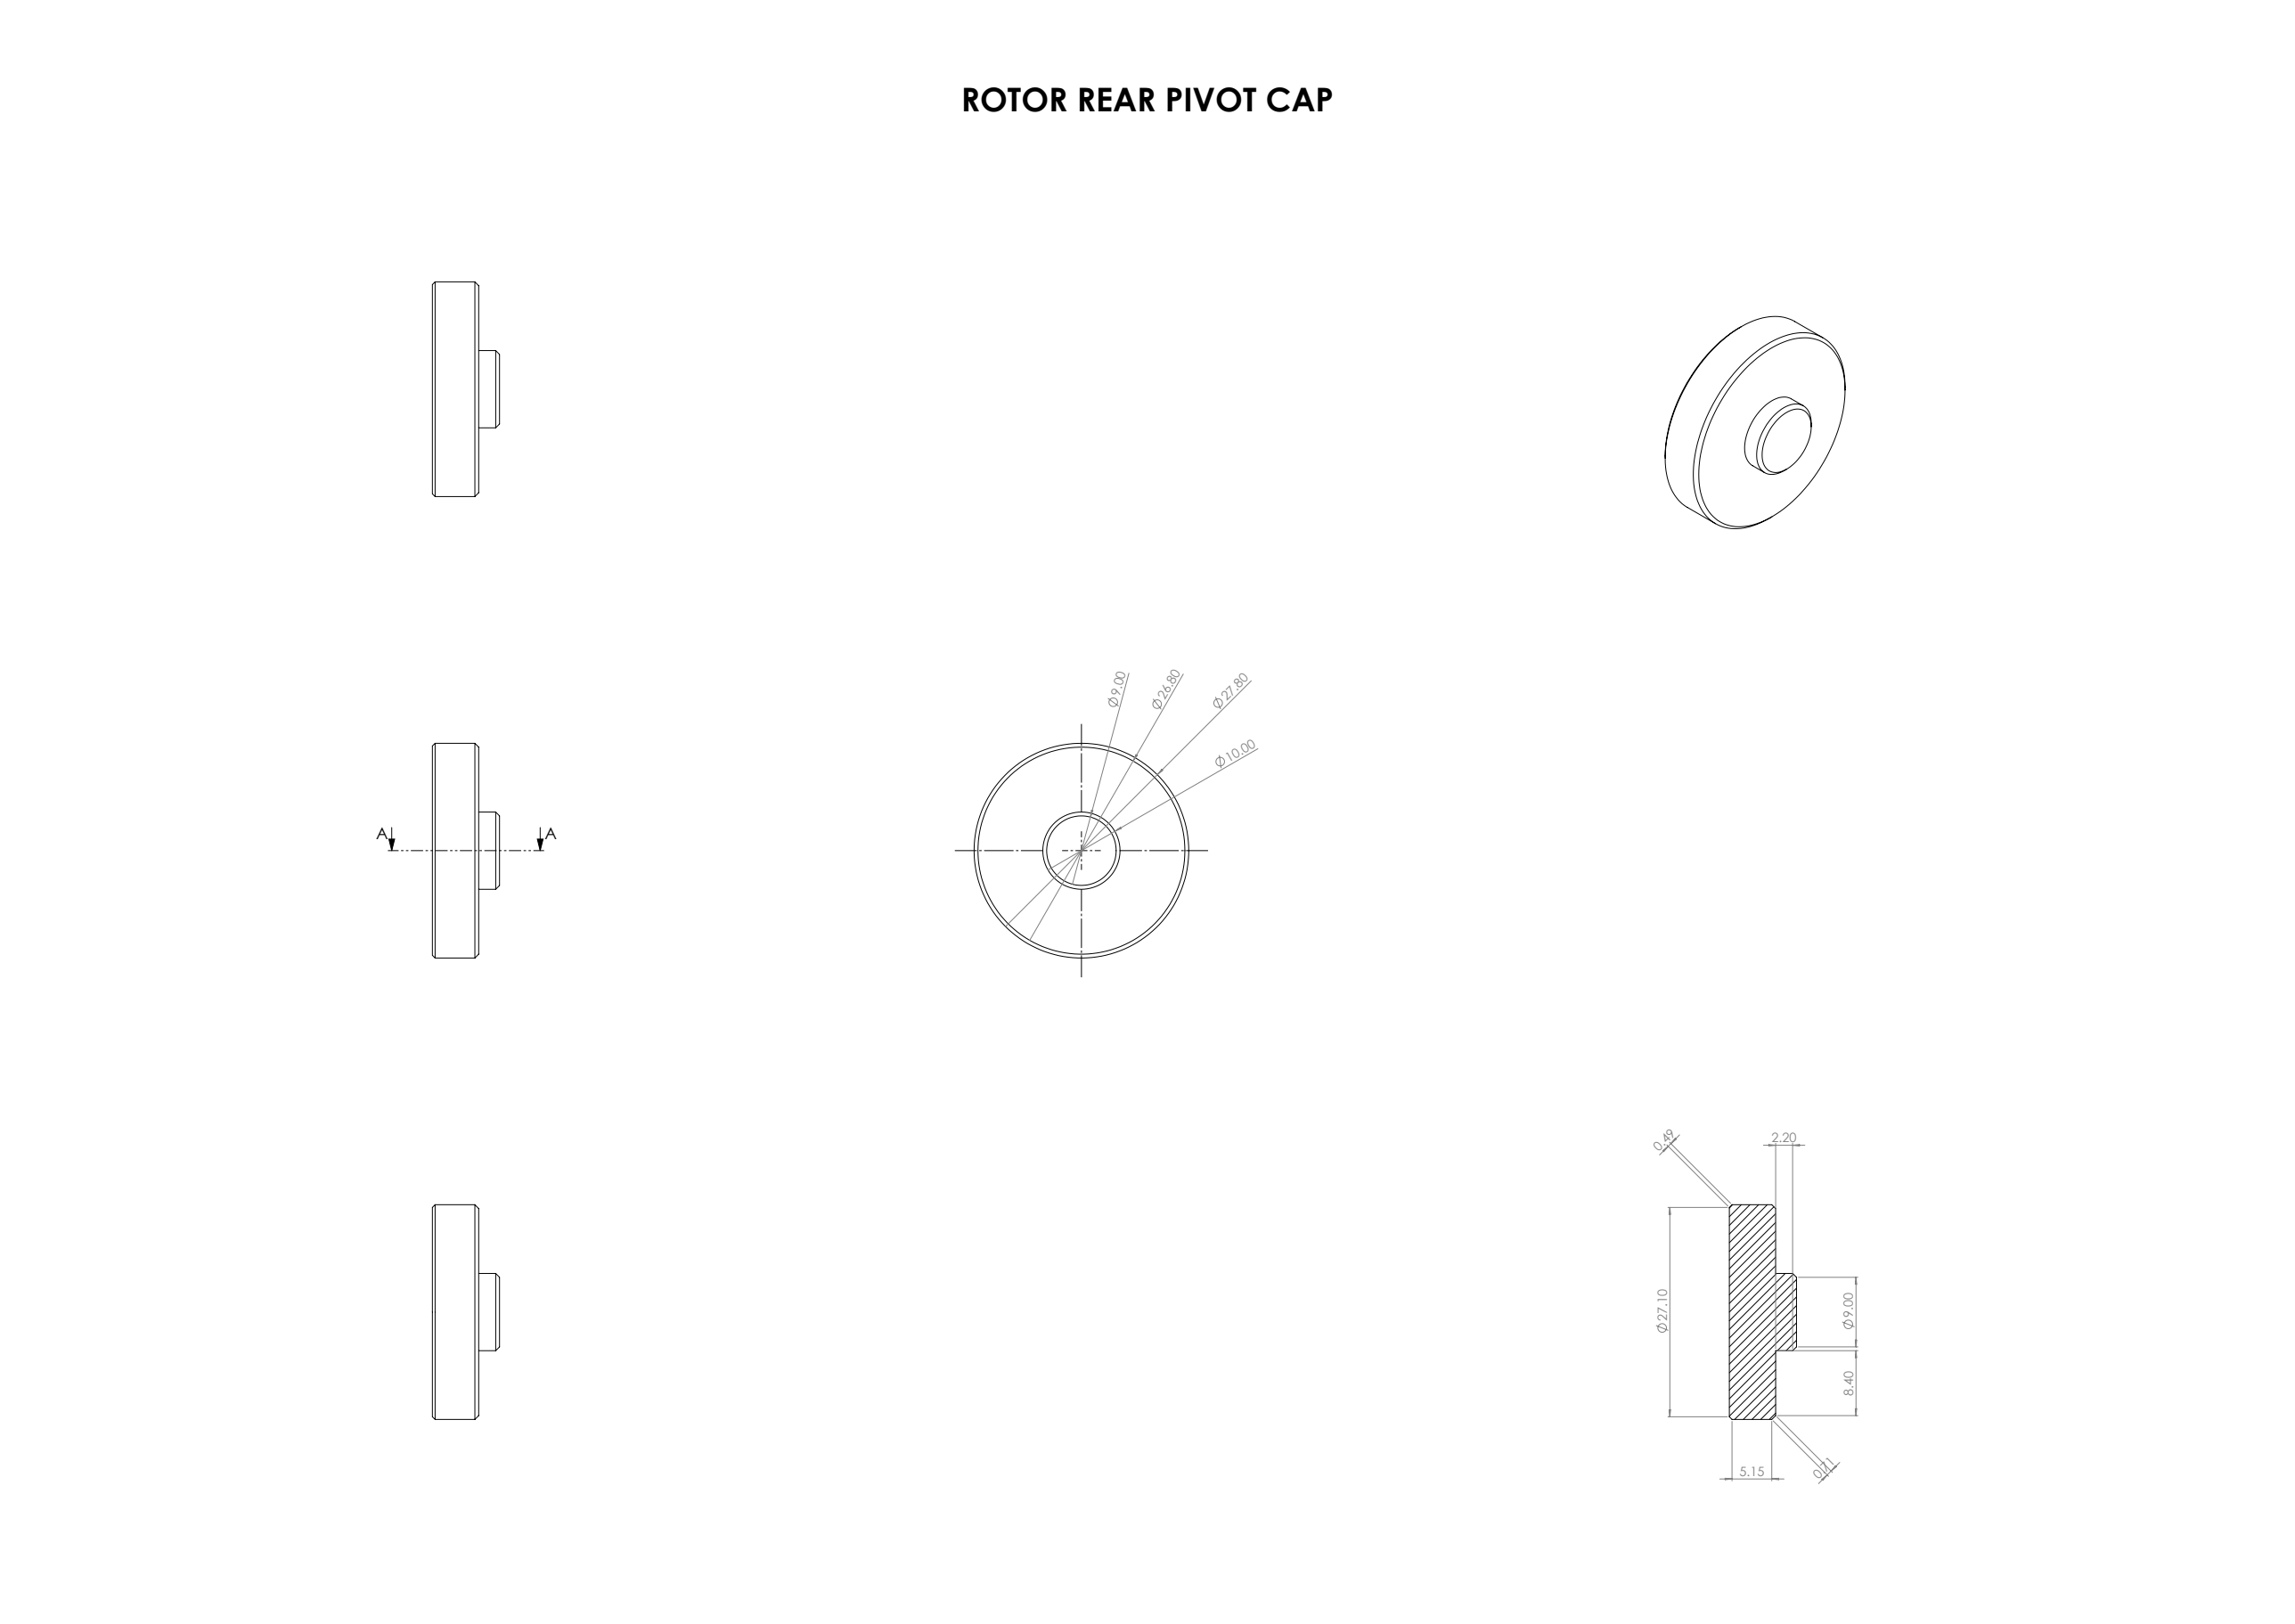
ISO-10303-21;
HEADER;
/* Generated by software containing ST-Developer
 * from STEP Tools, Inc. (www.steptools.com) 
 */

FILE_DESCRIPTION(
/* description */ (''),
/* implementation_level */ '2;1');

FILE_NAME(
/* name */ '05_Rotor_Rear_Pivot_Cap.step',
/* time_stamp */ '2026-10-21T01:59:45-07:00',
/* author */ (''),
/* organization */ (''),
/* preprocessor_version */ 'ST-DEVELOPER v20.2',
/* originating_system */ 'Autodesk Translation Framework v15.15.0.0',
/* authorisation */ '');

FILE_SCHEMA (('AUTOMOTIVE_DESIGN { 1 0 10303 214 3 1 1 }'));
ENDSEC;

DATA;
#10=MECHANICAL_DESIGN_GEOMETRIC_PRESENTATION_REPRESENTATION('',(#475),#18281);
#417=CONICAL_SURFACE('',#9697,13.725,0.785398163397447);
#418=CONICAL_SURFACE('',#9704,13.65,0.78539816339745);
#419=CONICAL_SURFACE('',#9710,4.75,0.785398163397449);
#444=SHAPE_REPRESENTATION_RELATIONSHIP('SRR','None',#18346,#457);
#457=ADVANCED_BREP_SHAPE_REPRESENTATION('',(#488),#18275);
#475=STYLED_ITEM('',(#18488),#488);
#488=MANIFOLD_SOLID_BREP('Body1',#9092);
#528=CYLINDRICAL_SURFACE('',#9702,13.9);
#529=CYLINDRICAL_SURFACE('',#9708,5.);
#619=FACE_BOUND('',#1765,.T.);
#747=CIRCLE('',#9698,13.9);
#748=CIRCLE('',#9699,13.9);
#749=CIRCLE('',#9700,13.55);
#750=CIRCLE('',#9703,13.9);
#751=CIRCLE('',#9705,13.4);
#752=CIRCLE('',#9707,5.);
#753=CIRCLE('',#9709,5.);
#754=CIRCLE('',#9711,4.5);
#1198=FACE_OUTER_BOUND('',#1760,.T.);
#1199=FACE_OUTER_BOUND('',#1761,.T.);
#1200=FACE_OUTER_BOUND('',#1762,.T.);
#1201=FACE_OUTER_BOUND('',#1763,.T.);
#1202=FACE_OUTER_BOUND('',#1764,.T.);
#1203=FACE_OUTER_BOUND('',#1766,.T.);
#1204=FACE_OUTER_BOUND('',#1767,.T.);
#1205=FACE_OUTER_BOUND('',#1768,.T.);
#1760=EDGE_LOOP('',(#7414,#7415,#7416,#7417,#7418));
#1761=EDGE_LOOP('',(#7419));
#1762=EDGE_LOOP('',(#7420,#7421,#7422,#7423,#7424));
#1763=EDGE_LOOP('',(#7425,#7426,#7427,#7428));
#1764=EDGE_LOOP('',(#7429));
#1765=EDGE_LOOP('',(#7430));
#1766=EDGE_LOOP('',(#7431,#7432,#7433,#7434));
#1767=EDGE_LOOP('',(#7435,#7436,#7437,#7438));
#1768=EDGE_LOOP('',(#7439));
#2562=LINE('',#14511,#3407);
#2563=LINE('',#14517,#3408);
#2564=LINE('',#14521,#3409);
#2565=LINE('',#14528,#3410);
#2566=LINE('',#14532,#3411);
#3407=VECTOR('',#11512,13.725);
#3408=VECTOR('',#11521,13.9);
#3409=VECTOR('',#11526,13.65);
#3410=VECTOR('',#11535,5.);
#3411=VECTOR('',#11540,4.75);
#4153=VERTEX_POINT('',#14506);
#4154=VERTEX_POINT('',#14507);
#4155=VERTEX_POINT('',#14510);
#4156=VERTEX_POINT('',#14515);
#4157=VERTEX_POINT('',#14519);
#4158=VERTEX_POINT('',#14523);
#4159=VERTEX_POINT('',#14526);
#4160=VERTEX_POINT('',#14530);
#5279=EDGE_CURVE('',#4153,#4154,#747,.T.);
#5280=EDGE_CURVE('',#4154,#4153,#748,.T.);
#5281=EDGE_CURVE('',#4153,#4155,#2562,.T.);
#5282=EDGE_CURVE('',#4155,#4155,#749,.T.);
#5283=EDGE_CURVE('',#4156,#4156,#750,.T.);
#5284=EDGE_CURVE('',#4156,#4154,#2563,.T.);
#5285=EDGE_CURVE('',#4157,#4157,#751,.T.);
#5286=EDGE_CURVE('',#4157,#4156,#2564,.T.);
#5287=EDGE_CURVE('',#4158,#4158,#752,.T.);
#5288=EDGE_CURVE('',#4159,#4159,#753,.T.);
#5289=EDGE_CURVE('',#4159,#4158,#2565,.T.);
#5290=EDGE_CURVE('',#4160,#4160,#754,.T.);
#5291=EDGE_CURVE('',#4160,#4159,#2566,.T.);
#7414=ORIENTED_EDGE('',*,*,#5279,.T.);
#7415=ORIENTED_EDGE('',*,*,#5280,.T.);
#7416=ORIENTED_EDGE('',*,*,#5281,.T.);
#7417=ORIENTED_EDGE('',*,*,#5282,.T.);
#7418=ORIENTED_EDGE('',*,*,#5281,.F.);
#7419=ORIENTED_EDGE('',*,*,#5282,.F.);
#7420=ORIENTED_EDGE('',*,*,#5283,.F.);
#7421=ORIENTED_EDGE('',*,*,#5284,.T.);
#7422=ORIENTED_EDGE('',*,*,#5279,.F.);
#7423=ORIENTED_EDGE('',*,*,#5280,.F.);
#7424=ORIENTED_EDGE('',*,*,#5284,.F.);
#7425=ORIENTED_EDGE('',*,*,#5285,.F.);
#7426=ORIENTED_EDGE('',*,*,#5286,.T.);
#7427=ORIENTED_EDGE('',*,*,#5283,.T.);
#7428=ORIENTED_EDGE('',*,*,#5286,.F.);
#7429=ORIENTED_EDGE('',*,*,#5285,.T.);
#7430=ORIENTED_EDGE('',*,*,#5287,.F.);
#7431=ORIENTED_EDGE('',*,*,#5288,.F.);
#7432=ORIENTED_EDGE('',*,*,#5289,.T.);
#7433=ORIENTED_EDGE('',*,*,#5287,.T.);
#7434=ORIENTED_EDGE('',*,*,#5289,.F.);
#7435=ORIENTED_EDGE('',*,*,#5290,.F.);
#7436=ORIENTED_EDGE('',*,*,#5291,.T.);
#7437=ORIENTED_EDGE('',*,*,#5288,.T.);
#7438=ORIENTED_EDGE('',*,*,#5291,.F.);
#7439=ORIENTED_EDGE('',*,*,#5290,.T.);
#8473=PLANE('',#9701);
#8474=PLANE('',#9706);
#8475=PLANE('',#9712);
#8919=ADVANCED_FACE('',(#1198),#417,.T.);
#8920=ADVANCED_FACE('',(#1199),#8473,.T.);
#8921=ADVANCED_FACE('',(#1200),#528,.T.);
#8922=ADVANCED_FACE('',(#1201),#418,.T.);
#8923=ADVANCED_FACE('',(#1202,#619),#8474,.T.);
#8924=ADVANCED_FACE('',(#1203),#529,.T.);
#8925=ADVANCED_FACE('',(#1204),#419,.T.);
#8926=ADVANCED_FACE('',(#1205),#8475,.T.);
#9092=CLOSED_SHELL('',(#8919,#8920,#8921,#8922,#8923,#8924,#8925,#8926));
#9696=AXIS2_PLACEMENT_3D('',#14504,#11504,#11505);
#9697=AXIS2_PLACEMENT_3D('',#14505,#11506,#11507);
#9698=AXIS2_PLACEMENT_3D('',#14508,#11508,#11509);
#9699=AXIS2_PLACEMENT_3D('',#14509,#11510,#11511);
#9700=AXIS2_PLACEMENT_3D('',#14512,#11513,#11514);
#9701=AXIS2_PLACEMENT_3D('',#14513,#11515,#11516);
#9702=AXIS2_PLACEMENT_3D('',#14514,#11517,#11518);
#9703=AXIS2_PLACEMENT_3D('',#14516,#11519,#11520);
#9704=AXIS2_PLACEMENT_3D('',#14518,#11522,#11523);
#9705=AXIS2_PLACEMENT_3D('',#14520,#11524,#11525);
#9706=AXIS2_PLACEMENT_3D('',#14522,#11527,#11528);
#9707=AXIS2_PLACEMENT_3D('',#14524,#11529,#11530);
#9708=AXIS2_PLACEMENT_3D('',#14525,#11531,#11532);
#9709=AXIS2_PLACEMENT_3D('',#14527,#11533,#11534);
#9710=AXIS2_PLACEMENT_3D('',#14529,#11536,#11537);
#9711=AXIS2_PLACEMENT_3D('',#14531,#11538,#11539);
#9712=AXIS2_PLACEMENT_3D('',#14533,#11541,#11542);
#11504=DIRECTION('axis',(0.,0.,1.));
#11505=DIRECTION('refdir',(1.,0.,0.));
#11506=DIRECTION('center_axis',(1.,0.,0.));
#11507=DIRECTION('ref_axis',(0.,-1.,0.));
#11508=DIRECTION('center_axis',(-1.,0.,0.));
#11509=DIRECTION('ref_axis',(0.,-1.,0.));
#11510=DIRECTION('center_axis',(-1.,0.,0.));
#11511=DIRECTION('ref_axis',(0.,-1.,0.));
#11512=DIRECTION('',(-0.707106781186548,-0.707106781186547,-8.65956056235492E-17));
#11513=DIRECTION('center_axis',(1.,0.,0.));
#11514=DIRECTION('ref_axis',(0.,-1.,0.));
#11515=DIRECTION('center_axis',(-1.,0.,0.));
#11516=DIRECTION('ref_axis',(0.,0.,1.));
#11517=DIRECTION('center_axis',(1.,0.,0.));
#11518=DIRECTION('ref_axis',(0.,1.,0.));
#11519=DIRECTION('center_axis',(1.,0.,0.));
#11520=DIRECTION('ref_axis',(0.,0.,-1.));
#11521=DIRECTION('',(-1.,0.,0.));
#11522=DIRECTION('center_axis',(-1.,0.,0.));
#11523=DIRECTION('ref_axis',(0.,1.,0.));
#11524=DIRECTION('center_axis',(1.,0.,0.));
#11525=DIRECTION('ref_axis',(0.,0.,-1.));
#11526=DIRECTION('',(-0.707106781186547,-0.707106781186548,-8.65956056235494E-17));
#11527=DIRECTION('center_axis',(1.,0.,0.));
#11528=DIRECTION('ref_axis',(0.,0.,-1.));
#11529=DIRECTION('center_axis',(1.,0.,0.));
#11530=DIRECTION('ref_axis',(0.,0.,-1.));
#11531=DIRECTION('center_axis',(1.,0.,0.));
#11532=DIRECTION('ref_axis',(0.,1.,0.));
#11533=DIRECTION('center_axis',(1.,0.,0.));
#11534=DIRECTION('ref_axis',(0.,0.,-1.));
#11535=DIRECTION('',(-1.,0.,0.));
#11536=DIRECTION('center_axis',(-1.,0.,0.));
#11537=DIRECTION('ref_axis',(0.,1.,0.));
#11538=DIRECTION('center_axis',(1.,0.,0.));
#11539=DIRECTION('ref_axis',(0.,0.,-1.));
#11540=DIRECTION('',(-0.707106781186547,-0.707106781186548,-8.65956056235494E-17));
#11541=DIRECTION('center_axis',(1.,0.,0.));
#11542=DIRECTION('ref_axis',(0.,0.,-1.));
#14504=CARTESIAN_POINT('',(0.,0.,0.));
#14505=CARTESIAN_POINT('Origin',(0.175,0.,0.));
#14506=CARTESIAN_POINT('',(0.35,13.9,-1.70225905081482E-15));
#14507=CARTESIAN_POINT('',(0.35,-13.9,-1.70225905081482E-15));
#14508=CARTESIAN_POINT('Origin',(0.35,0.,0.));
#14509=CARTESIAN_POINT('Origin',(0.35,0.,0.));
#14510=CARTESIAN_POINT('',(0.,13.55,1.65939641284466E-15));
#14511=CARTESIAN_POINT('',(0.175,13.725,1.68082773182974E-15));
#14512=CARTESIAN_POINT('Origin',(0.,0.,0.));
#14513=CARTESIAN_POINT('Origin',(0.,13.9,0.));
#14514=CARTESIAN_POINT('Origin',(2.75,0.,0.));
#14515=CARTESIAN_POINT('',(5.5,-13.9,-1.70225905081482E-15));
#14516=CARTESIAN_POINT('Origin',(5.5,0.,0.));
#14517=CARTESIAN_POINT('',(2.75,-13.9,-1.70225905081482E-15));
#14518=CARTESIAN_POINT('Origin',(5.75,0.,0.));
#14519=CARTESIAN_POINT('',(6.,-13.4,-1.64102671085745E-15));
#14520=CARTESIAN_POINT('Origin',(6.,0.,0.));
#14521=CARTESIAN_POINT('',(5.75,-13.65,-1.67164288083614E-15));
#14522=CARTESIAN_POINT('Origin',(6.,5.,0.));
#14523=CARTESIAN_POINT('',(6.,-5.,-6.12323399573677E-16));
#14524=CARTESIAN_POINT('Origin',(6.,0.,0.));
#14525=CARTESIAN_POINT('Origin',(7.1,0.,0.));
#14526=CARTESIAN_POINT('',(8.2,-5.,-6.12323399573677E-16));
#14527=CARTESIAN_POINT('Origin',(8.2,0.,0.));
#14528=CARTESIAN_POINT('',(7.1,-5.,-6.12323399573677E-16));
#14529=CARTESIAN_POINT('Origin',(8.45,0.,0.));
#14530=CARTESIAN_POINT('',(8.7,-4.5,-5.51091059616309E-16));
#14531=CARTESIAN_POINT('Origin',(8.7,0.,0.));
#14532=CARTESIAN_POINT('',(8.45,-4.75,-5.81707229594993E-16));
#14533=CARTESIAN_POINT('Origin',(8.7,0.,0.));
#18260=UNCERTAINTY_MEASURE_WITH_UNIT(LENGTH_MEASURE(0.01),#18282,
'DISTANCE_ACCURACY_VALUE',
'Maximum model space distance between geometric entities at asserted c
onnectivities');
#18266=UNCERTAINTY_MEASURE_WITH_UNIT(LENGTH_MEASURE(0.01),#18282,
'DISTANCE_ACCURACY_VALUE',
'Maximum model space distance between geometric entities at asserted c
onnectivities');
#18275=(
GEOMETRIC_REPRESENTATION_CONTEXT(3)
GLOBAL_UNCERTAINTY_ASSIGNED_CONTEXT((#18260))
GLOBAL_UNIT_ASSIGNED_CONTEXT((#18282,#18284,#18285))
REPRESENTATION_CONTEXT('','3D')
);
#18281=(
GEOMETRIC_REPRESENTATION_CONTEXT(3)
GLOBAL_UNCERTAINTY_ASSIGNED_CONTEXT((#18266))
GLOBAL_UNIT_ASSIGNED_CONTEXT((#18282,#18284,#18285))
REPRESENTATION_CONTEXT('','3D')
);
#18282=(
LENGTH_UNIT()
NAMED_UNIT(*)
SI_UNIT(.MILLI.,.METRE.)
);
#18284=(
NAMED_UNIT(*)
PLANE_ANGLE_UNIT()
SI_UNIT($,.RADIAN.)
);
#18285=(
NAMED_UNIT(*)
SI_UNIT($,.STERADIAN.)
SOLID_ANGLE_UNIT()
);
#18294=SHAPE_DEFINITION_REPRESENTATION(#18308,#18346);
#18308=PRODUCT_DEFINITION_SHAPE('',$,#18361);
#18346=SHAPE_REPRESENTATION('',(#9696),#18275);
#18352=PRODUCT_DEFINITION_CONTEXT('part definition',#18396,'design');
#18361=PRODUCT_DEFINITION('2026-10-20-13-03-18-806',
'05_Rotor_Rear_Pivot_Cap',#18375,#18352);
#18375=PRODUCT_DEFINITION_FORMATION('',$,#18406);
#18396=APPLICATION_CONTEXT(
'Core Data for Automotive Mechanical Design Process');
#18397=PRODUCT_CONTEXT('part definition',#18396,'mechanical');
#18406=PRODUCT('2026-10-20-13-03-18-806','05_Rotor_Rear_Pivot_Cap',$,(#18397));
#18482=COLOUR_RGB('Off White',0.89,0.88,0.83);
#18483=FILL_AREA_STYLE_COLOUR('',#18482);
#18484=FILL_AREA_STYLE('',(#18483));
#18485=SURFACE_STYLE_FILL_AREA(#18484);
#18486=SURFACE_SIDE_STYLE('',(#18485));
#18487=SURFACE_STYLE_USAGE(.BOTH.,#18486);
#18488=PRESENTATION_STYLE_ASSIGNMENT((#18487));
ENDSEC;
END-ISO-10303-21;
